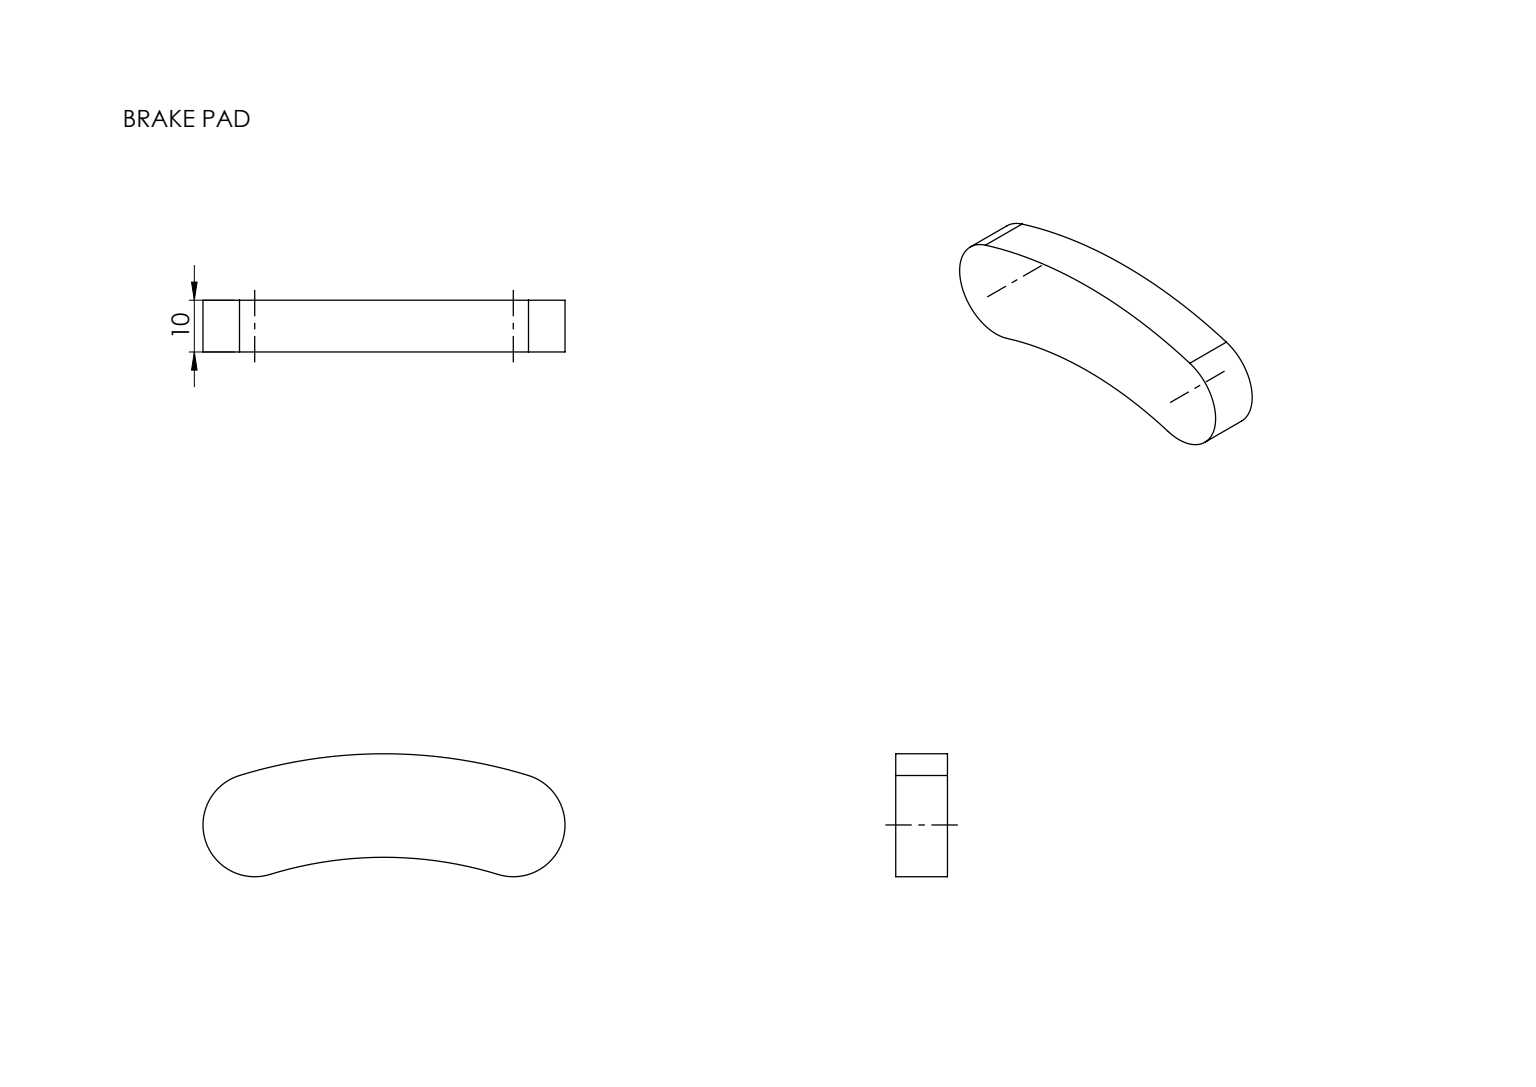
ISO-10303-21;
HEADER;
FILE_DESCRIPTION (('STEP AP214'),
    '1' );
FILE_NAME ('brake pad.step',
    '2026-10-02T06:35:35',
    ( '' ),
    ( '' ),
    'SwSTEP 2.0',
    'SolidWorks 2026',
    '' );
FILE_SCHEMA (( 'AUTOMOTIVE_DESIGN' ));
ENDSEC;

DATA;
#107=VECTOR ( 'NONE', #12064, 1000.000000000000000 ) ;
#177=ORIENTED_EDGE ( 'NONE', *, *, #5197, .F. ) ;
#226=ORIENTED_EDGE ( 'NONE', *, *, #3230, .T. ) ;
#296=CARTESIAN_POINT ( 'NONE',  ( 0.000000000000000000, 0.000000000000000000, 0.000000000000000000 ) ) ;
#385=AXIS2_PLACEMENT_3D ( 'NONE', #8772, #8688, #3163 ) ;
#389=DIRECTION ( 'NONE',  ( -1.000000000000000000, 0.000000000000000000, 0.000000000000000000 ) ) ;
#395=SURFACE_STYLE_USAGE ( .BOTH. , #9567 ) ;
#443=PLANE ( 'NONE',  #14295 ) ;
#460=( NAMED_UNIT ( * ) SI_UNIT ( $, .STERADIAN. ) SOLID_ANGLE_UNIT ( ) );
#479=VERTEX_POINT ( 'NONE', #11213 ) ;
#518=( LENGTH_UNIT ( ) NAMED_UNIT ( * ) SI_UNIT ( .MILLI., .METRE. ) );
#543=CARTESIAN_POINT ( 'NONE',  ( 0.000000000000000000, 0.000000000000000000, -23.50000000000000000 ) ) ;
#701=DIRECTION ( 'NONE',  ( -1.000000000000000000, 0.000000000000000000, 0.000000000000000000 ) ) ;
#750=SURFACE_SIDE_STYLE ('',( #10079 ) ) ;
#783=ORIENTED_EDGE ( 'NONE', *, *, #4911, .T. ) ;
#859=DIRECTION ( 'NONE',  ( 0.000000000000000000, 0.000000000000000000, -1.000000000000000000 ) ) ;
#879=VERTEX_POINT ( 'NONE', #11117 ) ;
#881=CIRCLE ( 'NONE', #5239, 10.00000000000000178 ) ;
#896=FACE_OUTER_BOUND ( 'NONE', #1263, .T. ) ;
#1026=PRODUCT_DEFINITION_SHAPE ( 'NONE', 'NONE',  #3579 ) ;
#1033=DIRECTION ( 'NONE',  ( 1.000000000000000000, 0.000000000000000000, 0.000000000000000000 ) ) ;
#1122=DIRECTION ( 'NONE',  ( -1.000000000000000000, 0.000000000000000000, 0.000000000000000000 ) ) ;
#1168=ADVANCED_FACE ( 'NONE', ( #2889 ), #14440, .F. ) ;
#1192=DIRECTION ( 'NONE',  ( -1.000000000000000000, 0.000000000000000000, 0.000000000000000000 ) ) ;
#1263=EDGE_LOOP ( 'NONE', ( #1616, #783, #4201, #4811 ) ) ;
#1335=AXIS2_PLACEMENT_3D ( 'NONE', #7355, #7432, #7205 ) ;
#1370=DIRECTION ( 'NONE',  ( 0.000000000000000000, 0.000000000000000000, -1.000000000000000000 ) ) ;
#1473=STYLED_ITEM ( 'NONE', ( #1754 ), #9171 ) ;
#1512=DIRECTION ( 'NONE',  ( 1.000000000000000000, 0.000000000000000000, 0.000000000000000000 ) ) ;
#1525=CARTESIAN_POINT ( 'NONE',  ( 0.000000000000000000, 0.000000000000000000, -13.50000000000000178 ) ) ;
#1541=DIRECTION ( 'NONE',  ( -1.000000000000000000, 0.000000000000000000, 0.000000000000000000 ) ) ;
#1557=AXIS2_PLACEMENT_3D ( 'NONE', #12081, #5164, #389 ) ;
#1602=DIRECTION ( 'NONE',  ( 0.000000000000000000, 0.000000000000000000, -1.000000000000000000 ) ) ;
#1610=FILL_AREA_STYLE ('',( #7286 ) ) ;
#1616=ORIENTED_EDGE ( 'NONE', *, *, #8934, .F. ) ;
#1704=EDGE_CURVE ( 'NONE', #4205, #10220, #881, .T. ) ;
#1754=PRESENTATION_STYLE_ASSIGNMENT (( #395 ) ) ;
#1841=ORIENTED_EDGE ( 'NONE', *, *, #1704, .T. ) ;
#1954=( NAMED_UNIT ( * ) SI_UNIT ( $, .STERADIAN. ) SOLID_ANGLE_UNIT ( ) );
#1965=ORIENTED_EDGE ( 'NONE', *, *, #11367, .F. ) ;
#1995=ADVANCED_FACE ( 'NONE', ( #896 ), #4080, .T. ) ;
#1996=ORIENTED_EDGE ( 'NONE', *, *, #8322, .T. ) ;
#2007=DIRECTION ( 'NONE',  ( 0.000000000000000000, 0.000000000000000000, -1.000000000000000000 ) ) ;
#2093=PRODUCT_CONTEXT ( 'NONE', #7647, 'mechanical' ) ;
#2121=CARTESIAN_POINT ( 'NONE',  ( -22.05882352941176450, 71.68269180561142662, -23.50000000000000000 ) ) ;
#2125=DIRECTION ( 'NONE',  ( -0.000000000000000000, -0.000000000000000000, 1.000000000000000000 ) ) ;
#2325=VERTEX_POINT ( 'NONE', #8825 ) ;
#2416=ORIENTED_EDGE ( 'NONE', *, *, #1704, .F. ) ;
#2434=( GEOMETRIC_REPRESENTATION_CONTEXT ( 3 ) GLOBAL_UNCERTAINTY_ASSIGNED_CONTEXT ( ( #8676 ) ) GLOBAL_UNIT_ASSIGNED_CONTEXT ( ( #6419, #14489, #1954 ) ) REPRESENTATION_CONTEXT ( 'NONE', 'WORKASPACE' ) );
#2602=EDGE_LOOP ( 'NONE', ( #2416, #1965, #8771, #177, #6324 ) ) ;
#2804=DIRECTION ( 'NONE',  ( -0.000000000000000000, -0.000000000000000000, 1.000000000000000000 ) ) ;
#2835=EDGE_LOOP ( 'NONE', ( #1841, #7715, #9592, #11283 ) ) ;
#2879=CARTESIAN_POINT ( 'NONE',  ( 35.00000000000000000, 81.24038404635960831, -13.50000000000000178 ) ) ;
#2889=FACE_OUTER_BOUND ( 'NONE', #8793, .T. ) ;
#2934=DIRECTION ( 'NONE',  ( -0.000000000000000000, -0.000000000000000000, 1.000000000000000000 ) ) ;
#2977=DIRECTION ( 'NONE',  ( -0.000000000000000000, -0.000000000000000000, 1.000000000000000000 ) ) ;
#3012=DIRECTION ( 'NONE',  ( -0.000000000000000000, -0.000000000000000000, 1.000000000000000000 ) ) ;
#3043=PRODUCT_DEFINITION_CONTEXT ( 'detailed design', #6968, 'design' ) ;
#3163=DIRECTION ( 'NONE',  ( 1.000000000000000000, 0.000000000000000000, 0.000000000000000000 ) ) ;
#3230=EDGE_CURVE ( 'NONE', #9159, #12354, #6712, .T. ) ;
#3235=ADVANCED_FACE ( 'NONE', ( #13333 ), #4239, .T. ) ;
#3277=ORIENTED_EDGE ( 'NONE', *, *, #5289, .F. ) ;
#3386=EDGE_CURVE ( 'NONE', #10213, #2325, #4674, .T. ) ;
#3429=AXIS2_PLACEMENT_3D ( 'NONE', #11606, #12742, #13652 ) ;
#3579=PRODUCT_DEFINITION ( 'UNKNOWN', '', #4853, #3043 ) ;
#3889=( NAMED_UNIT ( * ) PLANE_ANGLE_UNIT ( ) SI_UNIT ( $, .RADIAN. ) );
#3951=AXIS2_PLACEMENT_3D ( 'NONE', #10216, #14017, #1122 ) ;
#4017=SURFACE_STYLE_USAGE ( .BOTH. , #750 ) ;
#4080=CYLINDRICAL_SURFACE ( 'NONE', #385, 10.00000000000000178 ) ;
#4141=( GEOMETRIC_REPRESENTATION_CONTEXT ( 3 ) GLOBAL_UNCERTAINTY_ASSIGNED_CONTEXT ( ( #9733 ) ) GLOBAL_UNIT_ASSIGNED_CONTEXT ( ( #518, #7422, #9917 ) ) REPRESENTATION_CONTEXT ( 'NONE', 'WORKASPACE' ) );
#4172=SHAPE_REPRESENTATION_RELATIONSHIP ( 'NONE' , 'NONE' ,  #5964, #5117 ) ;
#4201=ORIENTED_EDGE ( 'NONE', *, *, #3386, .T. ) ;
#4205=VERTEX_POINT ( 'NONE', #9031 ) ;
#4239=CYLINDRICAL_SURFACE ( 'NONE', #11002, 10.00000000000000178 ) ;
#4466=VECTOR ( 'NONE', #2934, 1000.000000000000000 ) ;
#4674=CIRCLE ( 'NONE', #3951, 10.00000000000000355 ) ;
#4811=ORIENTED_EDGE ( 'NONE', *, *, #8322, .F. ) ;
#4844=VECTOR ( 'NONE', #2125, 1000.000000000000000 ) ;
#4853=PRODUCT_DEFINITION_FORMATION_WITH_SPECIFIED_SOURCE ( 'ANY', '', #11072, .NOT_KNOWN. ) ;
#4862=STYLED_ITEM ( 'NONE', ( #5378 ), #5117 ) ;
#4899=VECTOR ( 'NONE', #13900, 1000.000000000000000 ) ;
#4911=EDGE_CURVE ( 'NONE', #6576, #10213, #7415, .T. ) ;
#4952=ORIENTED_EDGE ( 'NONE', *, *, #11227, .T. ) ;
#5108=AXIS2_PLACEMENT_3D ( 'NONE', #296, #6125, #10768 ) ;
#5117=ADVANCED_BREP_SHAPE_REPRESENTATION ( '', ( #9171, #5108 ), #2434 ) ;
#5140=CIRCLE ( 'NONE', #12654, 10.00000000000000355 ) ;
#5164=DIRECTION ( 'NONE',  ( -0.000000000000000000, -0.000000000000000000, 1.000000000000000000 ) ) ;
#5197=EDGE_CURVE ( 'NONE', #12354, #10213, #8574, .T. ) ;
#5239=AXIS2_PLACEMENT_3D ( 'NONE', #8319, #12661, #1192 ) ;
#5278=ADVANCED_FACE ( 'NONE', ( #14600 ), #8811, .F. ) ;
#5281=CARTESIAN_POINT ( 'NONE',  ( 27.94117647058824616, 90.79807628710781842, -13.50000000000000178 ) ) ;
#5289=EDGE_CURVE ( 'NONE', #479, #879, #13433, .T. ) ;
#5378=PRESENTATION_STYLE_ASSIGNMENT (( #4017 ) ) ;
#5462=CIRCLE ( 'NONE', #10547, 10.00000000000000178 ) ;
#5499=VERTEX_POINT ( 'NONE', #5987 ) ;
#5582=VECTOR ( 'NONE', #8801, 1000.000000000000000 ) ;
#5788=FACE_OUTER_BOUND ( 'NONE', #2835, .T. ) ;
#5964=SHAPE_REPRESENTATION ( 'brake pad', ( #5108 ), #2434 ) ;
#5987=CARTESIAN_POINT ( 'NONE',  ( -27.94117647058823550, 90.79807628710781842, -23.50000000000000000 ) ) ;
#5990=CLOSED_SHELL ( 'NONE', ( #1995, #14046, #13063, #3235, #1168, #8390, #5278 ) ) ;
#6004=DIRECTION ( 'NONE',  ( 0.000000000000000000, 0.000000000000000000, -1.000000000000000000 ) ) ;
#6060=EDGE_CURVE ( 'NONE', #879, #5499, #5462, .T. ) ;
#6100=( GEOMETRIC_REPRESENTATION_CONTEXT ( 3 ) GLOBAL_UNCERTAINTY_ASSIGNED_CONTEXT ( ( #7728 ) ) GLOBAL_UNIT_ASSIGNED_CONTEXT ( ( #7505, #3889, #460 ) ) REPRESENTATION_CONTEXT ( 'NONE', 'WORKASPACE' ) );
#6125=DIRECTION ( 'NONE',  ( 0.000000000000000000, 0.000000000000000000, 1.000000000000000000 ) ) ;
#6267=DIRECTION ( 'NONE',  ( -1.000000000000000000, 0.000000000000000000, -0.000000000000000000 ) ) ;
#6324=ORIENTED_EDGE ( 'NONE', *, *, #10135, .F. ) ;
#6419=( LENGTH_UNIT ( ) NAMED_UNIT ( * ) SI_UNIT ( .MILLI., .METRE. ) );
#6452=CARTESIAN_POINT ( 'NONE',  ( 0.000000000000000000, 0.000000000000000000, -23.50000000000000000 ) ) ;
#6576=VERTEX_POINT ( 'NONE', #8058 ) ;
#6615=ORIENTED_EDGE ( 'NONE', *, *, #14715, .T. ) ;
#6668=LINE ( 'NONE', #12456, #5582 ) ;
#6708=ORIENTED_EDGE ( 'NONE', *, *, #11227, .F. ) ;
#6712=LINE ( 'NONE', #14779, #4466 ) ;
#6756=DIRECTION ( 'NONE',  ( -1.000000000000000000, 0.000000000000000000, 0.000000000000000000 ) ) ;
#6782=ORIENTED_EDGE ( 'NONE', *, *, #8673, .T. ) ;
#6874=AXIS2_PLACEMENT_3D ( 'NONE', #6452, #2977, #701 ) ;
#6892=LINE ( 'NONE', #2121, #4899 ) ;
#6968=APPLICATION_CONTEXT ( 'automotive_design' ) ;
#7035=MECHANICAL_DESIGN_GEOMETRIC_PRESENTATION_REPRESENTATION('',(#1473),#6100);
#7205=DIRECTION ( 'NONE',  ( -1.000000000000000000, 0.000000000000000000, 0.000000000000000000 ) ) ;
#7286=FILL_AREA_STYLE_COLOUR ( '', #10440 ) ;
#7355=CARTESIAN_POINT ( 'NONE',  ( 0.000000000000000000, 0.000000000000000000, -23.50000000000000000 ) ) ;
#7415=LINE ( 'NONE', #12408, #107 ) ;
#7422=( NAMED_UNIT ( * ) PLANE_ANGLE_UNIT ( ) SI_UNIT ( $, .RADIAN. ) );
#7432=DIRECTION ( 'NONE',  ( 0.000000000000000000, 0.000000000000000000, -1.000000000000000000 ) ) ;
#7505=( LENGTH_UNIT ( ) NAMED_UNIT ( * ) SI_UNIT ( .MILLI., .METRE. ) );
#7647=APPLICATION_CONTEXT ( 'automotive_design' ) ;
#7715=ORIENTED_EDGE ( 'NONE', *, *, #14715, .F. ) ;
#7728=UNCERTAINTY_MEASURE_WITH_UNIT (LENGTH_MEASURE( 1.000000000000000082E-05 ), #7505, 'distance_accuracy_value', 'NONE');
#7866=CIRCLE ( 'NONE', #1335, 95.00000000000001421 ) ;
#7930=EDGE_LOOP ( 'NONE', ( #10030, #12112, #226, #8263 ) ) ;
#7951=ORIENTED_EDGE ( 'NONE', *, *, #6060, .T. ) ;
#8058=CARTESIAN_POINT ( 'NONE',  ( 35.00000000000000000, 81.24038404635960831, -23.50000000000000000 ) ) ;
#8263=ORIENTED_EDGE ( 'NONE', *, *, #5197, .T. ) ;
#8319=CARTESIAN_POINT ( 'NONE',  ( -25.00000000000000000, 81.24038404635962252, -13.50000000000000178 ) ) ;
#8322=EDGE_CURVE ( 'NONE', #479, #2325, #10545, .T. ) ;
#8390=ADVANCED_FACE ( 'NONE', ( #9616 ), #443, .T. ) ;
#8426=DIRECTION ( 'NONE',  ( -1.000000000000000000, 0.000000000000000000, 0.000000000000000000 ) ) ;
#8483=CARTESIAN_POINT ( 'NONE',  ( -12.50000000000000000, 40.62019202317981126, -23.50000000000000000 ) ) ;
#8507=DIRECTION ( 'NONE',  ( -0.000000000000000000, -0.000000000000000000, 1.000000000000000000 ) ) ;
#8557=FACE_OUTER_BOUND ( 'NONE', #11384, .T. ) ;
#8574=CIRCLE ( 'NONE', #9537, 10.00000000000000355 ) ;
#8576=CARTESIAN_POINT ( 'NONE',  ( 27.94117647058824616, 90.79807628710781842, -23.50000000000000000 ) ) ;
#8673=EDGE_CURVE ( 'NONE', #9159, #6576, #13608, .T. ) ;
#8676=UNCERTAINTY_MEASURE_WITH_UNIT (LENGTH_MEASURE( 1.000000000000000082E-05 ), #6419, 'distance_accuracy_value', 'NONE');
#8688=DIRECTION ( 'NONE',  ( -0.000000000000000000, -0.000000000000000000, 1.000000000000000000 ) ) ;
#8771=ORIENTED_EDGE ( 'NONE', *, *, #3386, .F. ) ;
#8772=CARTESIAN_POINT ( 'NONE',  ( 25.00000000000000000, 81.24038404635960831, -23.50000000000000000 ) ) ;
#8793=EDGE_LOOP ( 'NONE', ( #11747, #13327, #3277, #1996 ) ) ;
#8801=DIRECTION ( 'NONE',  ( -0.000000000000000000, -0.000000000000000000, 1.000000000000000000 ) ) ;
#8811=PLANE ( 'NONE',  #12461 ) ;
#8825=CARTESIAN_POINT ( 'NONE',  ( 22.05882352941176094, 71.68269180561141241, -13.50000000000000178 ) ) ;
#8934=EDGE_CURVE ( 'NONE', #6576, #479, #5140, .T. ) ;
#9020=AXIS2_PLACEMENT_3D ( 'NONE', #9140, #10504, #1033 ) ;
#9031=CARTESIAN_POINT ( 'NONE',  ( -22.05882352941176450, 71.68269180561142662, -13.50000000000000178 ) ) ;
#9140=CARTESIAN_POINT ( 'NONE',  ( -25.00000000000000000, 81.24038404635962252, -23.50000000000000000 ) ) ;
#9159=VERTEX_POINT ( 'NONE', #8576 ) ;
#9171=MANIFOLD_SOLID_BREP ( 'Boss-Extrude1', #5990 ) ;
#9537=AXIS2_PLACEMENT_3D ( 'NONE', #9574, #6004, #1541 ) ;
#9544=CYLINDRICAL_SURFACE ( 'NONE', #11183, 95.00000000000001421 ) ;
#9567=SURFACE_SIDE_STYLE ('',( #10715 ) ) ;
#9574=CARTESIAN_POINT ( 'NONE',  ( 25.00000000000000000, 81.24038404635960831, -13.50000000000000178 ) ) ;
#9592=ORIENTED_EDGE ( 'NONE', *, *, #6060, .F. ) ;
#9616=FACE_OUTER_BOUND ( 'NONE', #13637, .T. ) ;
#9713=ORIENTED_EDGE ( 'NONE', *, *, #5289, .T. ) ;
#9733=UNCERTAINTY_MEASURE_WITH_UNIT (LENGTH_MEASURE( 1.000000000000000082E-05 ), #518, 'distance_accuracy_value', 'NONE');
#9868=ORIENTED_EDGE ( 'NONE', *, *, #8934, .T. ) ;
#9917=( NAMED_UNIT ( * ) SI_UNIT ( $, .STERADIAN. ) SOLID_ANGLE_UNIT ( ) );
#10028=ORIENTED_EDGE ( 'NONE', *, *, #10135, .T. ) ;
#10030=ORIENTED_EDGE ( 'NONE', *, *, #4911, .F. ) ;
#10079=SURFACE_STYLE_FILL_AREA ( #14725 ) ;
#10135=EDGE_CURVE ( 'NONE', #10220, #12354, #14310, .T. ) ;
#10191=AXIS2_PLACEMENT_3D ( 'NONE', #1525, #1602, #8426 ) ;
#10213=VERTEX_POINT ( 'NONE', #2879 ) ;
#10216=CARTESIAN_POINT ( 'NONE',  ( 25.00000000000000000, 81.24038404635960831, -13.50000000000000178 ) ) ;
#10220=VERTEX_POINT ( 'NONE', #12151 ) ;
#10440=COLOUR_RGB ( '', 0.40784314, 0.44705882, 0.49803922) ;
#10504=DIRECTION ( 'NONE',  ( -0.000000000000000000, -0.000000000000000000, 1.000000000000000000 ) ) ;
#10545=LINE ( 'NONE', #12535, #4844 ) ;
#10547=AXIS2_PLACEMENT_3D ( 'NONE', #12341, #2007, #13706 ) ;
#10715=SURFACE_STYLE_FILL_AREA ( #1610 ) ;
#10768=DIRECTION ( 'NONE',  ( 1.000000000000000000, 0.000000000000000000, 0.000000000000000000 ) ) ;
#10922=MECHANICAL_DESIGN_GEOMETRIC_PRESENTATION_REPRESENTATION('',(#4862),#4141);
#11002=AXIS2_PLACEMENT_3D ( 'NONE', #12350, #3012, #13636 ) ;
#11072=PRODUCT ( 'brake pad', 'brake pad', '', ( #2093 ) ) ;
#11117=CARTESIAN_POINT ( 'NONE',  ( -22.05882352941176450, 71.68269180561142662, -23.50000000000000000 ) ) ;
#11183=AXIS2_PLACEMENT_3D ( 'NONE', #14195, #2804, #1512 ) ;
#11213=CARTESIAN_POINT ( 'NONE',  ( 22.05882352941176094, 71.68269180561141241, -23.50000000000000000 ) ) ;
#11225=FILL_AREA_STYLE_COLOUR ( '', #13343 ) ;
#11227=EDGE_CURVE ( 'NONE', #5499, #9159, #7866, .T. ) ;
#11283=ORIENTED_EDGE ( 'NONE', *, *, #13735, .T. ) ;
#11287=SHAPE_DEFINITION_REPRESENTATION ( #1026, #5964 ) ;
#11367=EDGE_CURVE ( 'NONE', #2325, #4205, #14657, .T. ) ;
#11384=EDGE_LOOP ( 'NONE', ( #10028, #14631, #6708, #6615 ) ) ;
#11606=CARTESIAN_POINT ( 'NONE',  ( 25.00000000000000000, 81.24038404635960831, -23.50000000000000000 ) ) ;
#11747=ORIENTED_EDGE ( 'NONE', *, *, #11367, .T. ) ;
#12064=DIRECTION ( 'NONE',  ( -0.000000000000000000, -0.000000000000000000, 1.000000000000000000 ) ) ;
#12081=CARTESIAN_POINT ( 'NONE',  ( 0.000000000000000000, 0.000000000000000000, -13.50000000000000178 ) ) ;
#12112=ORIENTED_EDGE ( 'NONE', *, *, #8673, .F. ) ;
#12151=CARTESIAN_POINT ( 'NONE',  ( -27.94117647058823550, 90.79807628710781842, -13.50000000000000178 ) ) ;
#12341=CARTESIAN_POINT ( 'NONE',  ( -25.00000000000000000, 81.24038404635962252, -23.50000000000000000 ) ) ;
#12350=CARTESIAN_POINT ( 'NONE',  ( 25.00000000000000000, 81.24038404635960831, -23.50000000000000000 ) ) ;
#12354=VERTEX_POINT ( 'NONE', #5281 ) ;
#12408=CARTESIAN_POINT ( 'NONE',  ( 35.00000000000000000, 81.24038404635960831, -23.50000000000000000 ) ) ;
#12456=CARTESIAN_POINT ( 'NONE',  ( -27.94117647058823550, 90.79807628710781842, -23.50000000000000000 ) ) ;
#12461=AXIS2_PLACEMENT_3D ( 'NONE', #14445, #859, #13298 ) ;
#12535=CARTESIAN_POINT ( 'NONE',  ( 22.05882352941176094, 71.68269180561141241, -23.50000000000000000 ) ) ;
#12553=DIRECTION ( 'NONE',  ( 0.000000000000000000, 0.000000000000000000, -1.000000000000000000 ) ) ;
#12654=AXIS2_PLACEMENT_3D ( 'NONE', #14614, #12553, #6756 ) ;
#12661=DIRECTION ( 'NONE',  ( 0.000000000000000000, 0.000000000000000000, -1.000000000000000000 ) ) ;
#12742=DIRECTION ( 'NONE',  ( 0.000000000000000000, 0.000000000000000000, -1.000000000000000000 ) ) ;
#12858=CYLINDRICAL_SURFACE ( 'NONE', #9020, 10.00000000000000178 ) ;
#13063=ADVANCED_FACE ( 'NONE', ( #8557 ), #9544, .T. ) ;
#13176=AXIS2_PLACEMENT_3D ( 'NONE', #543, #8507, #13232 ) ;
#13232=DIRECTION ( 'NONE',  ( 1.000000000000000000, 0.000000000000000000, 0.000000000000000000 ) ) ;
#13298=DIRECTION ( 'NONE',  ( -1.000000000000000000, 0.000000000000000000, -0.000000000000000000 ) ) ;
#13327=ORIENTED_EDGE ( 'NONE', *, *, #13735, .F. ) ;
#13333=FACE_OUTER_BOUND ( 'NONE', #7930, .T. ) ;
#13343=COLOUR_RGB ( '', 0.40784314, 0.44705882, 0.49803922) ;
#13433=CIRCLE ( 'NONE', #6874, 75.00000000000001421 ) ;
#13608=CIRCLE ( 'NONE', #3429, 10.00000000000000355 ) ;
#13636=DIRECTION ( 'NONE',  ( 1.000000000000000000, 0.000000000000000000, 0.000000000000000000 ) ) ;
#13637=EDGE_LOOP ( 'NONE', ( #7951, #4952, #6782, #9868, #9713 ) ) ;
#13652=DIRECTION ( 'NONE',  ( -1.000000000000000000, 0.000000000000000000, 0.000000000000000000 ) ) ;
#13706=DIRECTION ( 'NONE',  ( -1.000000000000000000, 0.000000000000000000, 0.000000000000000000 ) ) ;
#13735=EDGE_CURVE ( 'NONE', #879, #4205, #6892, .T. ) ;
#13900=DIRECTION ( 'NONE',  ( -0.000000000000000000, -0.000000000000000000, 1.000000000000000000 ) ) ;
#14017=DIRECTION ( 'NONE',  ( 0.000000000000000000, 0.000000000000000000, -1.000000000000000000 ) ) ;
#14046=ADVANCED_FACE ( 'NONE', ( #5788 ), #12858, .T. ) ;
#14195=CARTESIAN_POINT ( 'NONE',  ( 0.000000000000000000, 0.000000000000000000, -23.50000000000000000 ) ) ;
#14295=AXIS2_PLACEMENT_3D ( 'NONE', #8483, #1370, #6267 ) ;
#14310=CIRCLE ( 'NONE', #10191, 95.00000000000001421 ) ;
#14440=CYLINDRICAL_SURFACE ( 'NONE', #13176, 75.00000000000001421 ) ;
#14445=CARTESIAN_POINT ( 'NONE',  ( -12.50000000000000000, 40.62019202317981126, -13.50000000000000178 ) ) ;
#14489=( NAMED_UNIT ( * ) PLANE_ANGLE_UNIT ( ) SI_UNIT ( $, .RADIAN. ) );
#14600=FACE_OUTER_BOUND ( 'NONE', #2602, .T. ) ;
#14614=CARTESIAN_POINT ( 'NONE',  ( 25.00000000000000000, 81.24038404635960831, -23.50000000000000000 ) ) ;
#14631=ORIENTED_EDGE ( 'NONE', *, *, #3230, .F. ) ;
#14657=CIRCLE ( 'NONE', #1557, 75.00000000000001421 ) ;
#14715=EDGE_CURVE ( 'NONE', #5499, #10220, #6668, .T. ) ;
#14725=FILL_AREA_STYLE ('',( #11225 ) ) ;
#14779=CARTESIAN_POINT ( 'NONE',  ( 27.94117647058824616, 90.79807628710781842, -23.50000000000000000 ) ) ;
ENDSEC;
END-ISO-10303-21;
